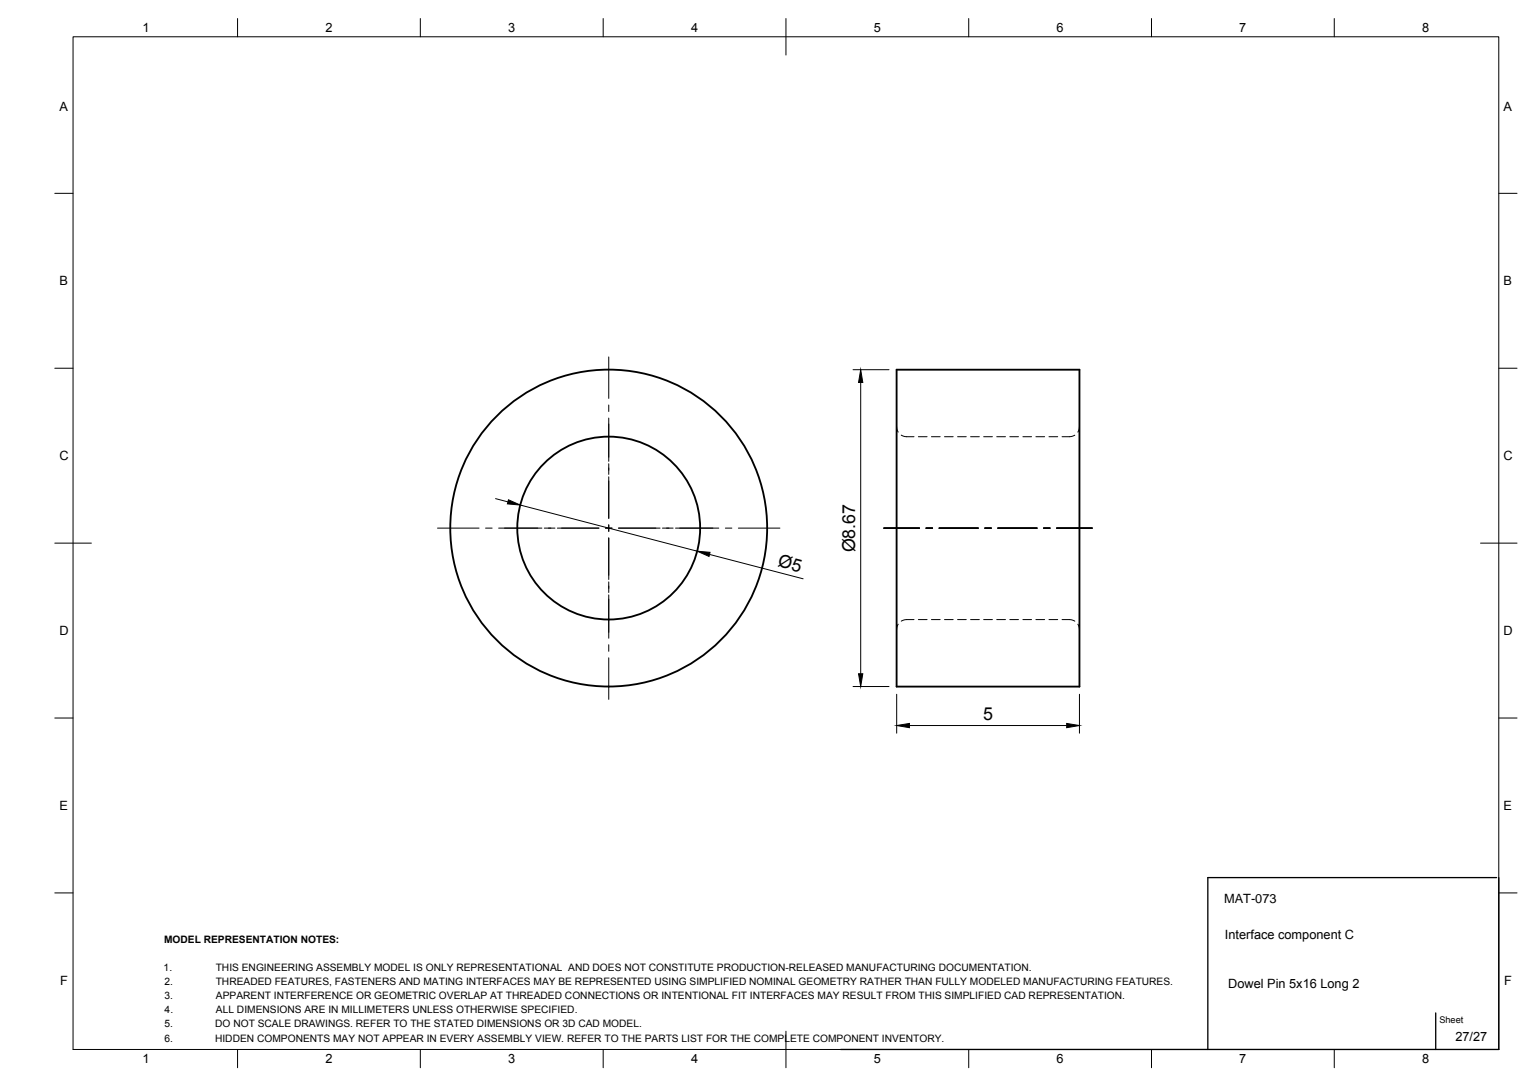
ISO-10303-21;
HEADER;
/* Generated by software containing ST-Developer
 * from STEP Tools, Inc. (www.steptools.com) 
 */

FILE_DESCRIPTION(
/* description */ ('CAx-IF Rec.Pracs.---Representation and Presentation of Product Manufa
cturing Information (PMI)---4.0---2014-10-13'),
/* implementation_level */ '2;1');

FILE_NAME(
/* name */ 'Interface component C.step',
/* time_stamp */ '2026-10-24T18:52:33-07:00',
/* author */ (''),
/* organization */ (''),
/* preprocessor_version */ 'ST-DEVELOPER v20.2',
/* originating_system */ 'Autodesk Translation Framework v15.17.0.0',
/* authorisation */ '');

FILE_SCHEMA (('AP242_MANAGED_MODEL_BASED_3D_ENGINEERING_MIM_LF { 1 0 10303 442 2 1 4 }'));
ENDSEC;

DATA;
#10=MECHANICAL_DESIGN_GEOMETRIC_PRESENTATION_REPRESENTATION('',(#444),#34876);
#378=SHAPE_REPRESENTATION_RELATIONSHIP('SRR','None',#35015,#411);
#411=ADVANCED_BREP_SHAPE_REPRESENTATION('',(#477),#34873);
#444=STYLED_ITEM('',(#35165),#477);
#477=MANIFOLD_SOLID_BREP('Dowel Pin 5x16 Long 2',#19584);
#586=FACE_BOUND('',#6947,.T.);
#587=FACE_BOUND('',#6950,.T.);
#1063=PLANE('',#22139);
#1064=PLANE('',#22144);
#2647=LINE('',#34359,#4246);
#2648=LINE('',#34372,#4247);
#4246=VECTOR('',#28196,0.0025);
#4247=VECTOR('',#28215,0.00433333333333334);
#4788=CYLINDRICAL_SURFACE('',#22136,0.0025);
#4789=CYLINDRICAL_SURFACE('',#22146,0.00433333333333334);
#5793=FACE_OUTER_BOUND('',#6944,.T.);
#5794=FACE_OUTER_BOUND('',#6945,.T.);
#5795=FACE_OUTER_BOUND('',#6946,.T.);
#5796=FACE_OUTER_BOUND('',#6948,.T.);
#5797=FACE_OUTER_BOUND('',#6949,.T.);
#5798=FACE_OUTER_BOUND('',#6951,.T.);
#6944=EDGE_LOOP('',(#18274,#18275,#18276,#18277,#18278));
#6945=EDGE_LOOP('',(#18279,#18280,#18281,#18282,#18283,#18284));
#6946=EDGE_LOOP('',(#18285));
#6947=EDGE_LOOP('',(#18286));
#6948=EDGE_LOOP('',(#18287,#18288,#18289,#18290,#18291));
#6949=EDGE_LOOP('',(#18292));
#6950=EDGE_LOOP('',(#18293));
#6951=EDGE_LOOP('',(#18294,#18295,#18296,#18297));
#8029=CIRCLE('',#22132,0.00250000000001);
#8030=CIRCLE('',#22133,0.000275);
#8031=CIRCLE('',#22134,0.00277500000001);
#8032=CIRCLE('',#22135,0.00250000000001);
#8033=CIRCLE('',#22137,0.00250000000001);
#8034=CIRCLE('',#22138,0.00250000000001);
#8035=CIRCLE('',#22140,0.00433333333334334);
#8036=CIRCLE('',#22142,0.00277500000001);
#8037=CIRCLE('',#22143,0.000275);
#8038=CIRCLE('',#22145,0.00433333333334334);
#9887=VERTEX_POINT('',#34348);
#9888=VERTEX_POINT('',#34349);
#9889=VERTEX_POINT('',#34351);
#9890=VERTEX_POINT('',#34356);
#9891=VERTEX_POINT('',#34357);
#9892=VERTEX_POINT('',#34362);
#9893=VERTEX_POINT('',#34365);
#9894=VERTEX_POINT('',#34369);
#12695=EDGE_CURVE('',#9887,#9888,#8029,.T.);
#12696=EDGE_CURVE('',#9888,#9889,#8030,.T.);
#12697=EDGE_CURVE('',#9889,#9889,#8031,.T.);
#12698=EDGE_CURVE('',#9888,#9887,#8032,.T.);
#12699=EDGE_CURVE('',#9890,#9891,#8033,.T.);
#12700=EDGE_CURVE('',#9890,#9887,#2647,.T.);
#12701=EDGE_CURVE('',#9891,#9890,#8034,.T.);
#12702=EDGE_CURVE('',#9892,#9892,#8035,.T.);
#12703=EDGE_CURVE('',#9893,#9893,#8036,.T.);
#12704=EDGE_CURVE('',#9893,#9891,#8037,.T.);
#12705=EDGE_CURVE('',#9894,#9894,#8038,.T.);
#12706=EDGE_CURVE('',#9892,#9894,#2648,.T.);
#18274=ORIENTED_EDGE('',*,*,#12695,.T.);
#18275=ORIENTED_EDGE('',*,*,#12696,.T.);
#18276=ORIENTED_EDGE('',*,*,#12697,.T.);
#18277=ORIENTED_EDGE('',*,*,#12696,.F.);
#18278=ORIENTED_EDGE('',*,*,#12698,.T.);
#18279=ORIENTED_EDGE('',*,*,#12699,.F.);
#18280=ORIENTED_EDGE('',*,*,#12700,.T.);
#18281=ORIENTED_EDGE('',*,*,#12698,.F.);
#18282=ORIENTED_EDGE('',*,*,#12695,.F.);
#18283=ORIENTED_EDGE('',*,*,#12700,.F.);
#18284=ORIENTED_EDGE('',*,*,#12701,.F.);
#18285=ORIENTED_EDGE('',*,*,#12702,.T.);
#18286=ORIENTED_EDGE('',*,*,#12697,.F.);
#18287=ORIENTED_EDGE('',*,*,#12703,.T.);
#18288=ORIENTED_EDGE('',*,*,#12704,.T.);
#18289=ORIENTED_EDGE('',*,*,#12701,.T.);
#18290=ORIENTED_EDGE('',*,*,#12699,.T.);
#18291=ORIENTED_EDGE('',*,*,#12704,.F.);
#18292=ORIENTED_EDGE('',*,*,#12705,.F.);
#18293=ORIENTED_EDGE('',*,*,#12703,.F.);
#18294=ORIENTED_EDGE('',*,*,#12702,.F.);
#18295=ORIENTED_EDGE('',*,*,#12706,.T.);
#18296=ORIENTED_EDGE('',*,*,#12705,.T.);
#18297=ORIENTED_EDGE('',*,*,#12706,.F.);
#18502=TOROIDAL_SURFACE('',#22131,0.002775,0.000275);
#18503=TOROIDAL_SURFACE('',#22141,0.002775,0.000275);
#19509=ADVANCED_FACE('',(#5793),#18502,.T.);
#19510=ADVANCED_FACE('',(#5794),#4788,.F.);
#19511=ADVANCED_FACE('',(#5795,#586),#1063,.T.);
#19512=ADVANCED_FACE('',(#5796),#18503,.T.);
#19513=ADVANCED_FACE('',(#5797,#587),#1064,.T.);
#19514=ADVANCED_FACE('',(#5798),#4789,.T.);
#19584=CLOSED_SHELL('',(#19509,#19510,#19511,#19512,#19513,#19514));
#22130=AXIS2_PLACEMENT_3D('',#34346,#28180,#28181);
#22131=AXIS2_PLACEMENT_3D('',#34347,#28182,#28183);
#22132=AXIS2_PLACEMENT_3D('',#34350,#28184,#28185);
#22133=AXIS2_PLACEMENT_3D('',#34352,#28186,#28187);
#22134=AXIS2_PLACEMENT_3D('',#34353,#28188,#28189);
#22135=AXIS2_PLACEMENT_3D('',#34354,#28190,#28191);
#22136=AXIS2_PLACEMENT_3D('',#34355,#28192,#28193);
#22137=AXIS2_PLACEMENT_3D('',#34358,#28194,#28195);
#22138=AXIS2_PLACEMENT_3D('',#34360,#28197,#28198);
#22139=AXIS2_PLACEMENT_3D('',#34361,#28199,#28200);
#22140=AXIS2_PLACEMENT_3D('',#34363,#28201,#28202);
#22141=AXIS2_PLACEMENT_3D('',#34364,#28203,#28204);
#22142=AXIS2_PLACEMENT_3D('',#34366,#28205,#28206);
#22143=AXIS2_PLACEMENT_3D('',#34367,#28207,#28208);
#22144=AXIS2_PLACEMENT_3D('',#34368,#28209,#28210);
#22145=AXIS2_PLACEMENT_3D('',#34370,#28211,#28212);
#22146=AXIS2_PLACEMENT_3D('',#34371,#28213,#28214);
#28180=DIRECTION('axis',(0.,0.,1.));
#28181=DIRECTION('refdir',(1.,0.,0.));
#28182=DIRECTION('center_axis',(4.55032717710333E-17,-1.,1.51850909121962E-32));
#28183=DIRECTION('ref_axis',(-0.770184521566975,0.,0.637821136948792));
#28184=DIRECTION('center_axis',(-4.55032717710333E-17,1.,-1.51850909121962E-32));
#28185=DIRECTION('ref_axis',(0.637821136951873,2.90229485360305E-17,0.770184521564424));
#28186=DIRECTION('center_axis',(0.637821136948792,2.90229485358903E-17,
0.770184521566975));
#28187=DIRECTION('ref_axis',(0.770184521566975,0.,-0.637821136948792));
#28188=DIRECTION('center_axis',(4.55032717710333E-17,-1.,1.51850909121962E-32));
#28189=DIRECTION('ref_axis',(0.637821136951568,2.90229485360166E-17,0.770184521564676));
#28190=DIRECTION('center_axis',(-4.55032717710333E-17,1.,-1.51850909121962E-32));
#28191=DIRECTION('ref_axis',(0.637821136951873,2.90229485360305E-17,0.770184521564424));
#28192=DIRECTION('center_axis',(4.55032717710333E-17,-1.,1.51850909121962E-32));
#28193=DIRECTION('ref_axis',(-0.637821136948792,-2.90229485358903E-17,-0.770184521566975));
#28194=DIRECTION('center_axis',(4.55032717710333E-17,-1.,1.51850909121962E-32));
#28195=DIRECTION('ref_axis',(0.637821136951873,2.90229485360305E-17,0.770184521564424));
#28196=DIRECTION('',(4.55032717710333E-17,-1.,1.51850909121962E-32));
#28197=DIRECTION('center_axis',(4.55032717710333E-17,-1.,1.51850909121962E-32));
#28198=DIRECTION('ref_axis',(0.637821136951873,2.90229485360305E-17,0.770184521564424));
#28199=DIRECTION('center_axis',(4.55032717710333E-17,-1.,1.51850909121962E-32));
#28200=DIRECTION('ref_axis',(-0.637821136948792,-2.90229485358903E-17,-0.770184521566975));
#28201=DIRECTION('center_axis',(4.55032717710333E-17,-1.,1.51850909121962E-32));
#28202=DIRECTION('ref_axis',(-0.637821136948792,-2.90229485358903E-17,-0.770184521566975));
#28203=DIRECTION('center_axis',(4.55032717710333E-17,-1.,1.51850909121962E-32));
#28204=DIRECTION('ref_axis',(-0.770184521566975,0.,0.637821136948792));
#28205=DIRECTION('center_axis',(-4.55032717710333E-17,1.,-1.51850909121962E-32));
#28206=DIRECTION('ref_axis',(0.637821136951568,2.90229485360166E-17,0.770184521564676));
#28207=DIRECTION('center_axis',(0.637821136948792,2.90229485358903E-17,
0.770184521566975));
#28208=DIRECTION('ref_axis',(0.770184521566975,0.,-0.637821136948792));
#28209=DIRECTION('center_axis',(-4.55032717710333E-17,1.,-1.51850909121962E-32));
#28210=DIRECTION('ref_axis',(0.770184521566975,3.50459155987053E-17,-0.637821136948792));
#28211=DIRECTION('center_axis',(4.55032717710333E-17,-1.,1.51850909121962E-32));
#28212=DIRECTION('ref_axis',(-0.637821136948792,-2.90229485358903E-17,-0.770184521566975));
#28213=DIRECTION('center_axis',(4.55032717710333E-17,-1.,1.51850909121962E-32));
#28214=DIRECTION('ref_axis',(-0.637821136948792,-2.90229485358903E-17,-0.770184521566975));
#28215=DIRECTION('',(-4.55032717710333E-17,1.,-1.51850909121962E-32));
#34346=CARTESIAN_POINT('',(0.,0.,0.));
#34347=CARTESIAN_POINT('Origin',(-4.50826289289608E-17,-0.006725,1.13636778952413E-32));
#34348=CARTESIAN_POINT('',(0.00159455284238602,-0.00672500000001,0.00192546130391876));
#34349=CARTESIAN_POINT('',(0.00192546130392509,-0.00672500000001,-0.00159455284237836));
#34350=CARTESIAN_POINT('Origin',(-4.50826289289603E-17,-0.00672500000001,
1.13636778952415E-32));
#34351=CARTESIAN_POINT('',(0.00213726204735601,-0.00700000000001,-0.00176995365503928));
#34352=CARTESIAN_POINT('Origin',(0.00213726204734831,-0.006725,-0.0017699536550329));
#34353=CARTESIAN_POINT('Origin',(-4.50701155292233E-17,-0.00700000000001,
1.13678537952423E-32));
#34354=CARTESIAN_POINT('Origin',(-4.50826289289603E-17,-0.00672500000001,
1.13636778952415E-32));
#34355=CARTESIAN_POINT('Origin',(-4.51838737086513E-17,-0.0045,1.13298910679617E-32));
#34356=CARTESIAN_POINT('',(0.00159455284238602,-0.00227500000001001,0.00192546130391876));
#34357=CARTESIAN_POINT('',(0.00192546130392509,-0.00227500000001001,-0.00159455284237836));
#34358=CARTESIAN_POINT('Origin',(-4.52851184883414E-17,-0.00227500000001001,
1.12961042406822E-32));
#34359=CARTESIAN_POINT('',(0.00159455284237193,-0.0045,0.00192546130391744));
#34360=CARTESIAN_POINT('Origin',(-4.52851184883414E-17,-0.00227500000001001,
1.12961042406822E-32));
#34361=CARTESIAN_POINT('Origin',(-0.00217922221790842,-0.007,-0.0026314637820205));
#34362=CARTESIAN_POINT('',(0.00276389159344472,-0.00700000000001,0.00333746626012356));
#34363=CARTESIAN_POINT('Origin',(-4.50701155292233E-17,-0.00700000000001,
1.13678537952423E-32));
#34364=CARTESIAN_POINT('Origin',(-4.52851184883419E-17,-0.002275,1.1296104240682E-32));
#34365=CARTESIAN_POINT('',(0.00213726204735601,-0.00200000000001001,-0.00176995365503928));
#34366=CARTESIAN_POINT('Origin',(-4.52976318880785E-17,-0.00200000000001001,
1.12919283406813E-32));
#34367=CARTESIAN_POINT('Origin',(0.00213726204734831,-0.002275,-0.0017699536550329));
#34368=CARTESIAN_POINT('Origin',(-0.00217922221790842,-0.002,-0.0026314637820205));
#34369=CARTESIAN_POINT('',(0.00276389159344472,-0.00200000000001001,0.00333746626012356));
#34370=CARTESIAN_POINT('Origin',(-4.52976318880785E-17,-0.00200000000001001,
1.12919283406813E-32));
#34371=CARTESIAN_POINT('Origin',(-4.51838737086513E-17,-0.0045,1.13298910679617E-32));
#34372=CARTESIAN_POINT('',(0.00276389159344472,-0.0045,0.00333746626012356));
#34838=UNCERTAINTY_MEASURE_WITH_UNIT(LENGTH_MEASURE(1.E-5),#34877,
'DISTANCE_ACCURACY_VALUE',
'Maximum model space distance between geometric entities at asserted c
onnectivities');
#34841=UNCERTAINTY_MEASURE_WITH_UNIT(LENGTH_MEASURE(1.E-5),#34877,
'DISTANCE_ACCURACY_VALUE',
'Maximum model space distance between geometric entities at asserted c
onnectivities');
#34873=(
GEOMETRIC_REPRESENTATION_CONTEXT(3)
GLOBAL_UNCERTAINTY_ASSIGNED_CONTEXT((#34838))
GLOBAL_UNIT_ASSIGNED_CONTEXT((#34877,#34878,#34879))
REPRESENTATION_CONTEXT('','3D')
);
#34876=(
GEOMETRIC_REPRESENTATION_CONTEXT(3)
GLOBAL_UNCERTAINTY_ASSIGNED_CONTEXT((#34841))
GLOBAL_UNIT_ASSIGNED_CONTEXT((#34877,#34878,#34879))
REPRESENTATION_CONTEXT('','3D')
);
#34877=(
LENGTH_UNIT()
NAMED_UNIT(*)
SI_UNIT($,.METRE.)
);
#34878=(
NAMED_UNIT(*)
PLANE_ANGLE_UNIT()
SI_UNIT($,.RADIAN.)
);
#34879=(
NAMED_UNIT(*)
SI_UNIT($,.STERADIAN.)
SOLID_ANGLE_UNIT()
);
#34911=SHAPE_DEFINITION_REPRESENTATION(#34945,#35015);
#34945=PRODUCT_DEFINITION_SHAPE('',$,#35050);
#35015=SHAPE_REPRESENTATION('',(#22130),#34873);
#35018=PRODUCT_DEFINITION_CONTEXT('part definition',#35122,'design');
#35050=PRODUCT_DEFINITION('Interface component C',
'Interface component C',#35084,#35018);
#35084=PRODUCT_DEFINITION_FORMATION('',$,#35155);
#35122=APPLICATION_CONTEXT('Managed model based 3d engineering');
#35123=PRODUCT_CONTEXT('part definition',#35122,'mechanical');
#35155=PRODUCT('Interface component C','Interface component C',
'LEGAL AND USAGE DISCLAIMER: this Data/Model is provided \X2\201C\X0\A
S IS\X2\201D\X0\ for informational and representational only. It is a 
geometric approximation and is NOT engineered, certified, or guarantee
d for dimensional accuracy, exact tolerances, or production-level prec
ision. Vendor disclaims all implied warranties including fitness for a
 particular purpose. DO NOT USE FOR DIRECT PHYSICAL MANUFACTURING, AUT
OMATED PRODUCTION, OR SAFETY-CRITICAL SYSTEMS without independent engi
neering verification and resolution of any design discrepancies.',(#35123));
#35165=PRESENTATION_STYLE_ASSIGNMENT((#35174));
#35174=SURFACE_STYLE_USAGE(.BOTH.,#35183);
#35183=SURFACE_SIDE_STYLE('',(#35192));
#35192=SURFACE_STYLE_FILL_AREA(#35201);
#35201=FILL_AREA_STYLE('Paint - Metallic (Blue)',(#35210));
#35210=FILL_AREA_STYLE_COLOUR('Paint - Metallic (Blue)',#35219);
#35219=COLOUR_RGB('Paint - Metallic (Blue)',0.188235294117647,0.231372549019608,
0.588235294117647);
ENDSEC;
END-ISO-10303-21;
